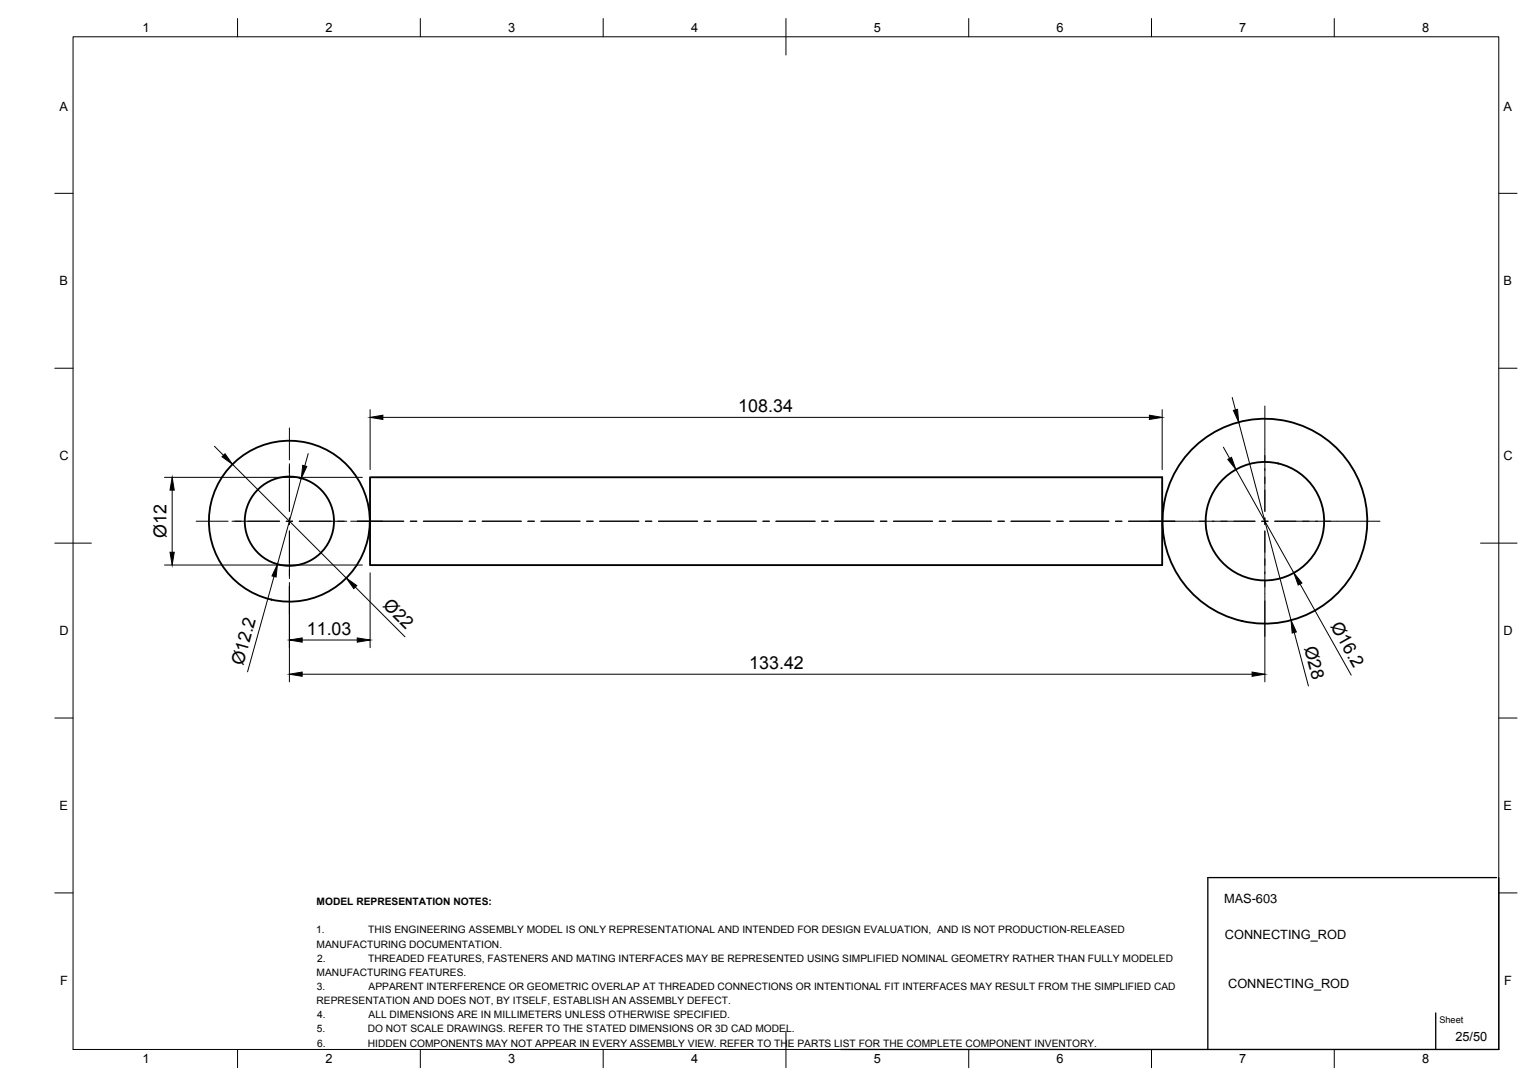
ISO-10303-21;
HEADER;
FILE_DESCRIPTION((''),'2;1');
FILE_NAME('CONNECTING_ROD.step','2026-10-01T22:06:14-07:00',(''),(''),'','','');
FILE_SCHEMA (('AUTOMOTIVE_DESIGN { 1 0 10303 214 3 1 1 }'));
ENDSEC;
DATA;
#10=MECHANICAL_DESIGN_GEOMETRIC_PRESENTATION_REPRESENTATION('',(#997,#998,#999),#50440);
#907=SHAPE_REPRESENTATION_RELATIONSHIP('SRR','None',#50639,#952) ;
#952=ADVANCED_BREP_SHAPE_REPRESENTATION('',(#1052,#1053,#1054),#50408) ;
#997=STYLED_ITEM('',(#50883),#1052) ;
#998=STYLED_ITEM('',(#50883),#1053) ;
#999=STYLED_ITEM('',(#50883),#1054) ;
#1052=MANIFOLD_SOLID_BREP('CONNECTING_ROD',#28664) ;
#1053=MANIFOLD_SOLID_BREP('CONNECTING_ROD',#28665) ;
#1054=MANIFOLD_SOLID_BREP('CONNECTING_ROD',#28666) ;
#1302=FACE_BOUND('',#4934,.T.) ;
#1303=FACE_BOUND('',#4936,.T.) ;
#1304=FACE_BOUND('',#4940,.T.) ;
#1305=FACE_BOUND('',#4942,.T.) ;
#2051=PLANE('',#30565) ;
#2052=PLANE('',#30566) ;
#2053=PLANE('',#30573) ;
#2054=PLANE('',#30574) ;
#2055=PLANE('',#30578) ;
#2056=PLANE('',#30579) ;
#3187=FACE_OUTER_BOUND('',#4931,.T.) ;
#3188=FACE_OUTER_BOUND('',#4932,.T.) ;
#3189=FACE_OUTER_BOUND('',#4933,.T.) ;
#3190=FACE_OUTER_BOUND('',#4935,.T.) ;
#3191=FACE_OUTER_BOUND('',#4937,.T.) ;
#3192=FACE_OUTER_BOUND('',#4938,.T.) ;
#3193=FACE_OUTER_BOUND('',#4939,.T.) ;
#3194=FACE_OUTER_BOUND('',#4941,.T.) ;
#3195=FACE_OUTER_BOUND('',#4943,.T.) ;
#3196=FACE_OUTER_BOUND('',#4944,.T.) ;
#3197=FACE_OUTER_BOUND('',#4945,.T.) ;
#4931=EDGE_LOOP('',(#22973,#22974,#22975,#22976)) ;
#4932=EDGE_LOOP('',(#22977,#22978,#22979,#22980)) ;
#4933=EDGE_LOOP('',(#22981)) ;
#4934=EDGE_LOOP('',(#22982)) ;
#4935=EDGE_LOOP('',(#22983)) ;
#4936=EDGE_LOOP('',(#22984)) ;
#4937=EDGE_LOOP('',(#22985,#22986,#22987,#22988)) ;
#4938=EDGE_LOOP('',(#22989,#22990,#22991,#22992)) ;
#4939=EDGE_LOOP('',(#22993)) ;
#4940=EDGE_LOOP('',(#22994)) ;
#4941=EDGE_LOOP('',(#22995)) ;
#4942=EDGE_LOOP('',(#22996)) ;
#4943=EDGE_LOOP('',(#22997,#22998,#22999,#23000)) ;
#4944=EDGE_LOOP('',(#23001)) ;
#4945=EDGE_LOOP('',(#23002)) ;
#7445=LINE('',#45920,#9917) ;
#7446=LINE('',#45926,#9918) ;
#7447=LINE('',#45934,#9919) ;
#7448=LINE('',#45940,#9920) ;
#7449=LINE('',#45948,#9921) ;
#9917=VECTOR('',#36792,0.61) ;
#9918=VECTOR('',#36799,1.1) ;
#9919=VECTOR('',#36810,0.81) ;
#9920=VECTOR('',#36817,1.4) ;
#9921=VECTOR('',#36828,0.6) ;
#11111=CIRCLE('',#30560,0.61) ;
#11112=CIRCLE('',#30561,0.61) ;
#11113=CIRCLE('',#30563,1.1) ;
#11114=CIRCLE('',#30564,1.1) ;
#11115=CIRCLE('',#30568,0.81) ;
#11116=CIRCLE('',#30569,0.81) ;
#11117=CIRCLE('',#30571,1.4) ;
#11118=CIRCLE('',#30572,1.4) ;
#11119=CIRCLE('',#30576,0.6) ;
#11120=CIRCLE('',#30577,0.6) ;
#13307=VERTEX_POINT('',#45917) ;
#13308=VERTEX_POINT('',#45919) ;
#13309=VERTEX_POINT('',#45923) ;
#13310=VERTEX_POINT('',#45925) ;
#13311=VERTEX_POINT('',#45931) ;
#13312=VERTEX_POINT('',#45933) ;
#13313=VERTEX_POINT('',#45937) ;
#13314=VERTEX_POINT('',#45939) ;
#13315=VERTEX_POINT('',#45945) ;
#13316=VERTEX_POINT('',#45947) ;
#16752=EDGE_CURVE('',#13307,#13307,#11111,.T.) ;
#16753=EDGE_CURVE('',#13307,#13308,#7445,.T.) ;
#16754=EDGE_CURVE('',#13308,#13308,#11112,.T.) ;
#16755=EDGE_CURVE('',#13309,#13309,#11113,.T.) ;
#16756=EDGE_CURVE('',#13309,#13310,#7446,.T.) ;
#16757=EDGE_CURVE('',#13310,#13310,#11114,.T.) ;
#16758=EDGE_CURVE('',#13311,#13311,#11115,.T.) ;
#16759=EDGE_CURVE('',#13311,#13312,#7447,.T.) ;
#16760=EDGE_CURVE('',#13312,#13312,#11116,.T.) ;
#16761=EDGE_CURVE('',#13313,#13313,#11117,.T.) ;
#16762=EDGE_CURVE('',#13313,#13314,#7448,.T.) ;
#16763=EDGE_CURVE('',#13314,#13314,#11118,.T.) ;
#16764=EDGE_CURVE('',#13315,#13315,#11119,.T.) ;
#16765=EDGE_CURVE('',#13315,#13316,#7449,.T.) ;
#16766=EDGE_CURVE('',#13316,#13316,#11120,.T.) ;
#22973=ORIENTED_EDGE('',*,*,#16752,.F.) ;
#22974=ORIENTED_EDGE('',*,*,#16753,.T.) ;
#22975=ORIENTED_EDGE('',*,*,#16754,.F.) ;
#22976=ORIENTED_EDGE('',*,*,#16753,.F.) ;
#22977=ORIENTED_EDGE('',*,*,#16755,.F.) ;
#22978=ORIENTED_EDGE('',*,*,#16756,.T.) ;
#22979=ORIENTED_EDGE('',*,*,#16757,.F.) ;
#22980=ORIENTED_EDGE('',*,*,#16756,.F.) ;
#22981=ORIENTED_EDGE('',*,*,#16757,.T.) ;
#22982=ORIENTED_EDGE('',*,*,#16752,.T.) ;
#22983=ORIENTED_EDGE('',*,*,#16755,.T.) ;
#22984=ORIENTED_EDGE('',*,*,#16754,.T.) ;
#22985=ORIENTED_EDGE('',*,*,#16758,.F.) ;
#22986=ORIENTED_EDGE('',*,*,#16759,.T.) ;
#22987=ORIENTED_EDGE('',*,*,#16760,.F.) ;
#22988=ORIENTED_EDGE('',*,*,#16759,.F.) ;
#22989=ORIENTED_EDGE('',*,*,#16761,.F.) ;
#22990=ORIENTED_EDGE('',*,*,#16762,.T.) ;
#22991=ORIENTED_EDGE('',*,*,#16763,.F.) ;
#22992=ORIENTED_EDGE('',*,*,#16762,.F.) ;
#22993=ORIENTED_EDGE('',*,*,#16763,.T.) ;
#22994=ORIENTED_EDGE('',*,*,#16758,.T.) ;
#22995=ORIENTED_EDGE('',*,*,#16761,.T.) ;
#22996=ORIENTED_EDGE('',*,*,#16760,.T.) ;
#22997=ORIENTED_EDGE('',*,*,#16764,.F.) ;
#22998=ORIENTED_EDGE('',*,*,#16765,.T.) ;
#22999=ORIENTED_EDGE('',*,*,#16766,.F.) ;
#23000=ORIENTED_EDGE('',*,*,#16765,.F.) ;
#23001=ORIENTED_EDGE('',*,*,#16766,.T.) ;
#23002=ORIENTED_EDGE('',*,*,#16764,.T.) ;
#26825=CYLINDRICAL_SURFACE('',#30559,0.61) ;
#26826=CYLINDRICAL_SURFACE('',#30562,1.1) ;
#26827=CYLINDRICAL_SURFACE('',#30567,0.81) ;
#26828=CYLINDRICAL_SURFACE('',#30570,1.4) ;
#26829=CYLINDRICAL_SURFACE('',#30575,0.6) ;
#27922=ADVANCED_FACE('',(#3187),#26825,.F.) ;
#27923=ADVANCED_FACE('',(#3188),#26826,.T.) ;
#27924=ADVANCED_FACE('',(#3189,#1302),#2051,.T.) ;
#27925=ADVANCED_FACE('',(#3190,#1303),#2052,.T.) ;
#27926=ADVANCED_FACE('',(#3191),#26827,.F.) ;
#27927=ADVANCED_FACE('',(#3192),#26828,.T.) ;
#27928=ADVANCED_FACE('',(#3193,#1304),#2053,.T.) ;
#27929=ADVANCED_FACE('',(#3194,#1305),#2054,.T.) ;
#27930=ADVANCED_FACE('',(#3195),#26829,.T.) ;
#27931=ADVANCED_FACE('',(#3196),#2055,.T.) ;
#27932=ADVANCED_FACE('',(#3197),#2056,.T.) ;
#28664=CLOSED_SHELL('',(#27922,#27923,#27924,#27925)) ;
#28665=CLOSED_SHELL('',(#27926,#27927,#27928,#27929)) ;
#28666=CLOSED_SHELL('',(#27930,#27931,#27932)) ;
#30558=AXIS2_PLACEMENT_3D('',#45915,#36786,#36787) ;
#30559=AXIS2_PLACEMENT_3D('',#45916,#36788,#36789) ;
#30560=AXIS2_PLACEMENT_3D('',#45918,#36790,#36791) ;
#30561=AXIS2_PLACEMENT_3D('',#45921,#36793,#36794) ;
#30562=AXIS2_PLACEMENT_3D('',#45922,#36795,#36796) ;
#30563=AXIS2_PLACEMENT_3D('',#45924,#36797,#36798) ;
#30564=AXIS2_PLACEMENT_3D('',#45927,#36800,#36801) ;
#30565=AXIS2_PLACEMENT_3D('',#45928,#36802,#36803) ;
#30566=AXIS2_PLACEMENT_3D('',#45929,#36804,#36805) ;
#30567=AXIS2_PLACEMENT_3D('',#45930,#36806,#36807) ;
#30568=AXIS2_PLACEMENT_3D('',#45932,#36808,#36809) ;
#30569=AXIS2_PLACEMENT_3D('',#45935,#36811,#36812) ;
#30570=AXIS2_PLACEMENT_3D('',#45936,#36813,#36814) ;
#30571=AXIS2_PLACEMENT_3D('',#45938,#36815,#36816) ;
#30572=AXIS2_PLACEMENT_3D('',#45941,#36818,#36819) ;
#30573=AXIS2_PLACEMENT_3D('',#45942,#36820,#36821) ;
#30574=AXIS2_PLACEMENT_3D('',#45943,#36822,#36823) ;
#30575=AXIS2_PLACEMENT_3D('',#45944,#36824,#36825) ;
#30576=AXIS2_PLACEMENT_3D('',#45946,#36826,#36827) ;
#30577=AXIS2_PLACEMENT_3D('',#45949,#36829,#36830) ;
#30578=AXIS2_PLACEMENT_3D('',#45950,#36831,#36832) ;
#30579=AXIS2_PLACEMENT_3D('',#45951,#36833,#36834) ;
#36786=DIRECTION('axis',(0.,0.,1.)) ;
#36787=DIRECTION('refdir',(1.,0.,0.)) ;
#36788=DIRECTION('center_axis',(0.,1.,0.)) ;
#36789=DIRECTION('ref_axis',(1.,0.,0.)) ;
#36790=DIRECTION('center_axis',(0.,1.,0.)) ;
#36791=DIRECTION('ref_axis',(1.,0.,0.)) ;
#36792=DIRECTION('',(0.,1.,0.)) ;
#36793=DIRECTION('center_axis',(0.,-1.,0.)) ;
#36794=DIRECTION('ref_axis',(1.,0.,0.)) ;
#36795=DIRECTION('center_axis',(0.,1.,0.)) ;
#36796=DIRECTION('ref_axis',(1.,0.,0.)) ;
#36797=DIRECTION('center_axis',(0.,1.,0.)) ;
#36798=DIRECTION('ref_axis',(1.,0.,0.)) ;
#36799=DIRECTION('',(0.,-1.,0.)) ;
#36800=DIRECTION('center_axis',(0.,-1.,0.)) ;
#36801=DIRECTION('ref_axis',(1.,0.,0.)) ;
#36802=DIRECTION('center_axis',(0.,-1.,0.)) ;
#36803=DIRECTION('ref_axis',(-1.,0.,0.)) ;
#36804=DIRECTION('center_axis',(0.,1.,0.)) ;
#36805=DIRECTION('ref_axis',(1.,0.,0.)) ;
#36806=DIRECTION('center_axis',(0.,1.,0.)) ;
#36807=DIRECTION('ref_axis',(1.,0.,0.)) ;
#36808=DIRECTION('center_axis',(0.,1.,0.)) ;
#36809=DIRECTION('ref_axis',(1.,0.,0.)) ;
#36810=DIRECTION('',(0.,1.,0.)) ;
#36811=DIRECTION('center_axis',(0.,-1.,0.)) ;
#36812=DIRECTION('ref_axis',(1.,0.,0.)) ;
#36813=DIRECTION('center_axis',(0.,1.,0.)) ;
#36814=DIRECTION('ref_axis',(1.,0.,0.)) ;
#36815=DIRECTION('center_axis',(0.,1.,0.)) ;
#36816=DIRECTION('ref_axis',(1.,0.,0.)) ;
#36817=DIRECTION('',(0.,-1.,0.)) ;
#36818=DIRECTION('center_axis',(0.,-1.,0.)) ;
#36819=DIRECTION('ref_axis',(1.,0.,0.)) ;
#36820=DIRECTION('center_axis',(0.,-1.,0.)) ;
#36821=DIRECTION('ref_axis',(-1.,0.,0.)) ;
#36822=DIRECTION('center_axis',(0.,1.,0.)) ;
#36823=DIRECTION('ref_axis',(1.,0.,0.)) ;
#36824=DIRECTION('center_axis',(-0.224859506698758,0.,-0.97439119569462)) ;
#36825=DIRECTION('ref_axis',(0.97439119569462,0.,-0.224859506698758)) ;
#36826=DIRECTION('center_axis',(-0.224859506698758,0.,-0.97439119569462)) ;
#36827=DIRECTION('ref_axis',(0.97439119569462,0.,-0.224859506698758)) ;
#36828=DIRECTION('',(0.224859506698758,0.,0.97439119569462)) ;
#36829=DIRECTION('center_axis',(0.224859506698758,0.,0.97439119569462)) ;
#36830=DIRECTION('ref_axis',(0.97439119569462,0.,-0.224859506698758)) ;
#36831=DIRECTION('center_axis',(0.224859506698758,0.,0.97439119569462)) ;
#36832=DIRECTION('ref_axis',(-0.97439119569462,0.,0.224859506698758)) ;
#36833=DIRECTION('center_axis',(-0.224859506698758,0.,-0.97439119569462)) ;
#36834=DIRECTION('ref_axis',(0.97439119569462,0.,-0.224859506698758)) ;
#45915=CARTESIAN_POINT('',(0.,0.,0.)) ;
#45916=CARTESIAN_POINT('Origin',(0.,-15.7,24.)) ;
#45917=CARTESIAN_POINT('',(-0.61,-16.2,24.)) ;
#45918=CARTESIAN_POINT('Origin',(0.,-16.2,24.)) ;
#45919=CARTESIAN_POINT('',(-0.61,-15.2,24.)) ;
#45920=CARTESIAN_POINT('',(-0.61,-15.7,24.)) ;
#45921=CARTESIAN_POINT('Origin',(0.,-15.2,24.)) ;
#45922=CARTESIAN_POINT('Origin',(0.,-15.7,24.)) ;
#45923=CARTESIAN_POINT('',(-1.1,-15.2,24.)) ;
#45924=CARTESIAN_POINT('Origin',(0.,-15.2,24.)) ;
#45925=CARTESIAN_POINT('',(-1.1,-16.2,24.)) ;
#45926=CARTESIAN_POINT('',(-1.1,-15.7,24.)) ;
#45927=CARTESIAN_POINT('Origin',(0.,-16.2,24.)) ;
#45928=CARTESIAN_POINT('Origin',(0.,-16.2,24.)) ;
#45929=CARTESIAN_POINT('Origin',(0.,-15.2,24.)) ;
#45930=CARTESIAN_POINT('Origin',(3.,-15.7,37.)) ;
#45931=CARTESIAN_POINT('',(2.19,-16.2,37.)) ;
#45932=CARTESIAN_POINT('Origin',(3.,-16.2,37.)) ;
#45933=CARTESIAN_POINT('',(2.19,-15.2,37.)) ;
#45934=CARTESIAN_POINT('',(2.19,-15.7,37.)) ;
#45935=CARTESIAN_POINT('Origin',(3.,-15.2,37.)) ;
#45936=CARTESIAN_POINT('Origin',(3.,-15.7,37.)) ;
#45937=CARTESIAN_POINT('',(1.6,-15.2,37.)) ;
#45938=CARTESIAN_POINT('Origin',(3.,-15.2,37.)) ;
#45939=CARTESIAN_POINT('',(1.6,-16.2,37.)) ;
#45940=CARTESIAN_POINT('',(1.6,-15.7,37.)) ;
#45941=CARTESIAN_POINT('Origin',(3.,-16.2,37.)) ;
#45942=CARTESIAN_POINT('Origin',(3.,-16.2,37.)) ;
#45943=CARTESIAN_POINT('Origin',(3.,-15.2,37.)) ;
#45944=CARTESIAN_POINT('Origin',(1.46616541353383,-15.7,30.3533834586466)) ;
#45945=CARTESIAN_POINT('',(-0.336514416664893,-15.7,25.2101036739441)) ;
#45946=CARTESIAN_POINT('Origin',(0.24812030075188,-15.7,25.0751879699248)) ;
#45947=CARTESIAN_POINT('',(2.09957580889902,-15.7,35.7664946513877)) ;
#45948=CARTESIAN_POINT('',(0.881530696117062,-15.7,30.4882991626659)) ;
#45949=CARTESIAN_POINT('Origin',(2.68421052631579,-15.7,35.6315789473684)) ;
#45950=CARTESIAN_POINT('Origin',(2.68421052631579,-15.7,35.6315789473684)) ;
#45951=CARTESIAN_POINT('Origin',(0.24812030075188,-15.7,25.0751879699248)) ;
#50355=UNCERTAINTY_MEASURE_WITH_UNIT(LENGTH_MEASURE(0.001),#50441,
'DISTANCE_ACCURACY_VALUE',
'Maximum model space distance between geometric entities at asserted c
onnectivities') ;
#50387=UNCERTAINTY_MEASURE_WITH_UNIT(LENGTH_MEASURE(0.001),#50441,
'DISTANCE_ACCURACY_VALUE',
'Maximum model space distance between geometric entities at asserted c
onnectivities') ;
#50408=(
GEOMETRIC_REPRESENTATION_CONTEXT(3)
GLOBAL_UNCERTAINTY_ASSIGNED_CONTEXT((#50355))
GLOBAL_UNIT_ASSIGNED_CONTEXT((#50441,#50443,#50444))
REPRESENTATION_CONTEXT('','3D')
) ;
#50440=(
GEOMETRIC_REPRESENTATION_CONTEXT(3)
GLOBAL_UNCERTAINTY_ASSIGNED_CONTEXT((#50387))
GLOBAL_UNIT_ASSIGNED_CONTEXT((#50441,#50443,#50444))
REPRESENTATION_CONTEXT('','3D')
) ;
#50441=(
LENGTH_UNIT()
NAMED_UNIT(*)
SI_UNIT(.CENTI.,.METRE.)
) ;
#50443=(
NAMED_UNIT(*)
PLANE_ANGLE_UNIT()
SI_UNIT($,.RADIAN.)
) ;
#50444=(
NAMED_UNIT(*)
SI_UNIT($,.STERADIAN.)
SOLID_ANGLE_UNIT()
) ;
#50465=SHAPE_DEFINITION_REPRESENTATION(#50531,#50639) ;
#50531=PRODUCT_DEFINITION_SHAPE('',$,#50692) ;
#50639=SHAPE_REPRESENTATION('',(#30558),#50408) ;
#50671=PRODUCT_DEFINITION_CONTEXT('part definition',#50829,'design') ;
#50692=PRODUCT_DEFINITION('CONNECTING_ROD','CONNECTING_ROD',#50744,
#50671) ;
#50744=PRODUCT_DEFINITION_FORMATION('',$,#50851) ;
#50829=APPLICATION_CONTEXT(
'Core Data for Automotive Mechanical Design Process') ;
#50830=PRODUCT_CONTEXT('part definition',#50829,'mechanical') ;
#50851=PRODUCT('CONNECTING_ROD','CONNECTING_ROD',$,(#50830)) ;
#50883=PRESENTATION_STYLE_ASSIGNMENT((#50890)) ;
#50890=SURFACE_STYLE_USAGE(.BOTH.,#50897) ;
#50897=SURFACE_SIDE_STYLE('',(#50904)) ;
#50904=SURFACE_STYLE_FILL_AREA(#50911) ;
#50911=FILL_AREA_STYLE('Steel - Satin',(#50918)) ;
#50918=FILL_AREA_STYLE_COLOUR('Steel - Satin',#50925) ;
#50925=COLOUR_RGB('Steel - Satin', 0.31764706, 0.68627451, 0.89019608) ;
ENDSEC;
END-ISO-10303-21;
